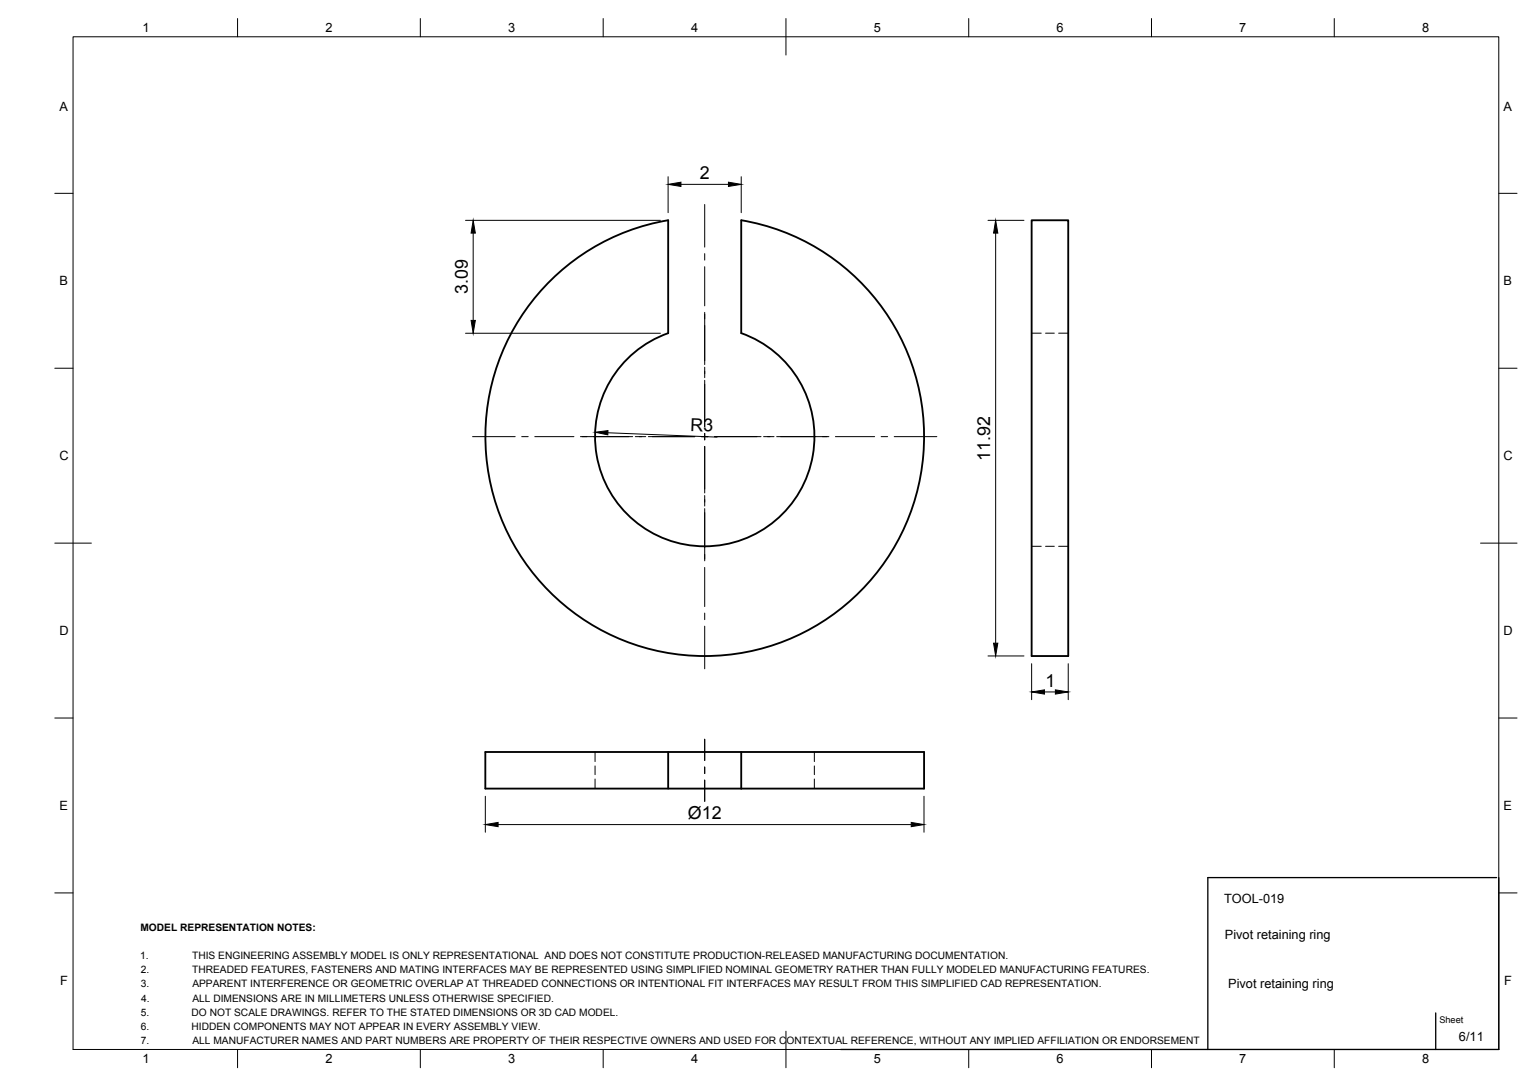
ISO-10303-21;
HEADER;
/* Generated by software containing ST-Developer
 * from STEP Tools, Inc. (www.steptools.com) 
 */

FILE_DESCRIPTION(
/* description */ (''),
/* implementation_level */ '2;1');

FILE_NAME(
/* name */ 'Pivot retaining ring.step',
/* time_stamp */ '2026-11-10T09:14:46-08:00',
/* author */ (''),
/* organization */ (''),
/* preprocessor_version */ 'ST-DEVELOPER v20.2',
/* originating_system */ 'Autodesk Translation Framework v15.17.0.0',
/* authorisation */ '');

FILE_SCHEMA (('AUTOMOTIVE_DESIGN { 1 0 10303 214 3 1 1 }'));
ENDSEC;

DATA;
#10=MECHANICAL_DESIGN_GEOMETRIC_PRESENTATION_REPRESENTATION('',(#561),#19471);
#541=SHAPE_REPRESENTATION_RELATIONSHIP('SRR','None',#19520,#551);
#551=ADVANCED_BREP_SHAPE_REPRESENTATION('',(#571),#19463);
#561=STYLED_ITEM('',(#19583),#571);
#571=MANIFOLD_SOLID_BREP('Body1',#7154);
#702=PLANE('',#7412);
#703=PLANE('',#7413);
#704=PLANE('',#7414);
#705=PLANE('',#7421);
#897=FACE_OUTER_BOUND('',#1325,.T.);
#898=FACE_OUTER_BOUND('',#1326,.T.);
#899=FACE_OUTER_BOUND('',#1327,.T.);
#900=FACE_OUTER_BOUND('',#1328,.T.);
#901=FACE_OUTER_BOUND('',#1329,.T.);
#902=FACE_OUTER_BOUND('',#1330,.T.);
#1325=EDGE_LOOP('',(#4925,#4926,#4927,#4928));
#1326=EDGE_LOOP('',(#4929,#4930,#4931,#4932));
#1327=EDGE_LOOP('',(#4933,#4934,#4935,#4936));
#1328=EDGE_LOOP('',(#4937,#4938,#4939,#4940));
#1329=EDGE_LOOP('',(#4941,#4942,#4943,#4944));
#1330=EDGE_LOOP('',(#4945,#4946,#4947,#4948));
#1843=LINE('',#9788,#2317);
#1844=LINE('',#9790,#2318);
#1845=LINE('',#9792,#2319);
#1846=LINE('',#9793,#2320);
#1847=LINE('',#9797,#2321);
#1848=LINE('',#9799,#2322);
#1849=LINE('',#9801,#2323);
#1850=LINE('',#9802,#2324);
#2317=VECTOR('',#8235,1.);
#2318=VECTOR('',#8236,1.);
#2319=VECTOR('',#8237,1.);
#2320=VECTOR('',#8238,1.);
#2321=VECTOR('',#8241,1.);
#2322=VECTOR('',#8242,1.);
#2323=VECTOR('',#8243,1.);
#2324=VECTOR('',#8244,1.);
#2715=CIRCLE('',#7415,0.6);
#2716=CIRCLE('',#7416,0.3);
#2717=CIRCLE('',#7418,0.3);
#2718=CIRCLE('',#7420,0.6);
#2971=VERTEX_POINT('',#9786);
#2972=VERTEX_POINT('',#9787);
#2973=VERTEX_POINT('',#9789);
#2974=VERTEX_POINT('',#9791);
#2975=VERTEX_POINT('',#9795);
#2976=VERTEX_POINT('',#9796);
#2977=VERTEX_POINT('',#9798);
#2978=VERTEX_POINT('',#9800);
#3703=EDGE_CURVE('',#2971,#2972,#1843,.T.);
#3704=EDGE_CURVE('',#2973,#2971,#1844,.T.);
#3705=EDGE_CURVE('',#2974,#2973,#1845,.T.);
#3706=EDGE_CURVE('',#2972,#2974,#1846,.T.);
#3707=EDGE_CURVE('',#2975,#2976,#1847,.T.);
#3708=EDGE_CURVE('',#2977,#2975,#1848,.T.);
#3709=EDGE_CURVE('',#2978,#2977,#1849,.T.);
#3710=EDGE_CURVE('',#2976,#2978,#1850,.T.);
#3711=EDGE_CURVE('',#2973,#2978,#2715,.T.);
#3712=EDGE_CURVE('',#2976,#2971,#2716,.T.);
#3713=EDGE_CURVE('',#2975,#2972,#2717,.T.);
#3714=EDGE_CURVE('',#2974,#2977,#2718,.T.);
#4925=ORIENTED_EDGE('',*,*,#3703,.F.);
#4926=ORIENTED_EDGE('',*,*,#3704,.F.);
#4927=ORIENTED_EDGE('',*,*,#3705,.F.);
#4928=ORIENTED_EDGE('',*,*,#3706,.F.);
#4929=ORIENTED_EDGE('',*,*,#3707,.F.);
#4930=ORIENTED_EDGE('',*,*,#3708,.F.);
#4931=ORIENTED_EDGE('',*,*,#3709,.F.);
#4932=ORIENTED_EDGE('',*,*,#3710,.F.);
#4933=ORIENTED_EDGE('',*,*,#3710,.T.);
#4934=ORIENTED_EDGE('',*,*,#3711,.F.);
#4935=ORIENTED_EDGE('',*,*,#3704,.T.);
#4936=ORIENTED_EDGE('',*,*,#3712,.F.);
#4937=ORIENTED_EDGE('',*,*,#3707,.T.);
#4938=ORIENTED_EDGE('',*,*,#3712,.T.);
#4939=ORIENTED_EDGE('',*,*,#3703,.T.);
#4940=ORIENTED_EDGE('',*,*,#3713,.F.);
#4941=ORIENTED_EDGE('',*,*,#3709,.T.);
#4942=ORIENTED_EDGE('',*,*,#3714,.F.);
#4943=ORIENTED_EDGE('',*,*,#3705,.T.);
#4944=ORIENTED_EDGE('',*,*,#3711,.T.);
#4945=ORIENTED_EDGE('',*,*,#3708,.T.);
#4946=ORIENTED_EDGE('',*,*,#3713,.T.);
#4947=ORIENTED_EDGE('',*,*,#3706,.T.);
#4948=ORIENTED_EDGE('',*,*,#3714,.T.);
#6625=CYLINDRICAL_SURFACE('',#7417,0.3);
#6626=CYLINDRICAL_SURFACE('',#7419,0.6);
#6819=ADVANCED_FACE('',(#897),#702,.F.);
#6820=ADVANCED_FACE('',(#898),#703,.F.);
#6821=ADVANCED_FACE('',(#899),#704,.F.);
#6822=ADVANCED_FACE('',(#900),#6625,.F.);
#6823=ADVANCED_FACE('',(#901),#6626,.T.);
#6824=ADVANCED_FACE('',(#902),#705,.T.);
#7154=CLOSED_SHELL('',(#6819,#6820,#6821,#6822,#6823,#6824));
#7411=AXIS2_PLACEMENT_3D('',#9784,#8231,#8232);
#7412=AXIS2_PLACEMENT_3D('',#9785,#8233,#8234);
#7413=AXIS2_PLACEMENT_3D('',#9794,#8239,#8240);
#7414=AXIS2_PLACEMENT_3D('',#9803,#8245,#8246);
#7415=AXIS2_PLACEMENT_3D('',#9804,#8247,#8248);
#7416=AXIS2_PLACEMENT_3D('',#9805,#8249,#8250);
#7417=AXIS2_PLACEMENT_3D('',#9806,#8251,#8252);
#7418=AXIS2_PLACEMENT_3D('',#9807,#8253,#8254);
#7419=AXIS2_PLACEMENT_3D('',#9808,#8255,#8256);
#7420=AXIS2_PLACEMENT_3D('',#9809,#8257,#8258);
#7421=AXIS2_PLACEMENT_3D('',#9810,#8259,#8260);
#8231=DIRECTION('axis',(0.,0.,1.));
#8232=DIRECTION('refdir',(1.,0.,0.));
#8233=DIRECTION('center_axis',(-1.,0.,0.));
#8234=DIRECTION('ref_axis',(0.,1.,0.));
#8235=DIRECTION('',(0.,0.,1.));
#8236=DIRECTION('',(0.,-1.,0.));
#8237=DIRECTION('',(0.,0.,-1.));
#8238=DIRECTION('',(0.,1.,0.));
#8239=DIRECTION('center_axis',(1.,0.,0.));
#8240=DIRECTION('ref_axis',(0.,-1.,0.));
#8241=DIRECTION('',(0.,0.,-1.));
#8242=DIRECTION('',(0.,-1.,0.));
#8243=DIRECTION('',(0.,0.,1.));
#8244=DIRECTION('',(0.,1.,0.));
#8245=DIRECTION('center_axis',(0.,0.,1.));
#8246=DIRECTION('ref_axis',(1.,0.,0.));
#8247=DIRECTION('center_axis',(0.,0.,1.));
#8248=DIRECTION('ref_axis',(1.,0.,0.));
#8249=DIRECTION('center_axis',(0.,0.,-1.));
#8250=DIRECTION('ref_axis',(1.,0.,0.));
#8251=DIRECTION('center_axis',(0.,0.,1.));
#8252=DIRECTION('ref_axis',(6.12323399573677E-17,-1.,0.));
#8253=DIRECTION('center_axis',(0.,0.,-1.));
#8254=DIRECTION('ref_axis',(1.,0.,0.));
#8255=DIRECTION('center_axis',(0.,0.,1.));
#8256=DIRECTION('ref_axis',(6.12323399573677E-17,-1.,0.));
#8257=DIRECTION('center_axis',(0.,0.,1.));
#8258=DIRECTION('ref_axis',(1.,0.,0.));
#8259=DIRECTION('center_axis',(0.,0.,1.));
#8260=DIRECTION('ref_axis',(1.,0.,0.));
#9784=CARTESIAN_POINT('',(0.,0.,0.));
#9785=CARTESIAN_POINT('Origin',(-0.1,0.,0.1));
#9786=CARTESIAN_POINT('',(-0.1,0.282842712474619,0.));
#9787=CARTESIAN_POINT('',(-0.1,0.282842712474619,0.1));
#9788=CARTESIAN_POINT('',(-0.1,0.282842712474619,0.));
#9789=CARTESIAN_POINT('',(-0.1,0.591607978309962,0.));
#9790=CARTESIAN_POINT('',(-0.1,0.,0.));
#9791=CARTESIAN_POINT('',(-0.1,0.591607978309962,0.1));
#9792=CARTESIAN_POINT('',(-0.1,0.591607978309962,0.));
#9793=CARTESIAN_POINT('',(-0.1,0.,0.1));
#9794=CARTESIAN_POINT('Origin',(0.1,1.2,0.1));
#9795=CARTESIAN_POINT('',(0.1,0.282842712474619,0.1));
#9796=CARTESIAN_POINT('',(0.1,0.282842712474619,0.));
#9797=CARTESIAN_POINT('',(0.1,0.282842712474619,0.));
#9798=CARTESIAN_POINT('',(0.1,0.591607978309962,0.1));
#9799=CARTESIAN_POINT('',(0.1,0.6,0.1));
#9800=CARTESIAN_POINT('',(0.1,0.591607978309962,0.));
#9801=CARTESIAN_POINT('',(0.1,0.591607978309962,0.));
#9802=CARTESIAN_POINT('',(0.1,0.6,0.));
#9803=CARTESIAN_POINT('Origin',(0.,0.,0.));
#9804=CARTESIAN_POINT('Origin',(0.,0.,0.));
#9805=CARTESIAN_POINT('Origin',(0.,0.,0.));
#9806=CARTESIAN_POINT('Origin',(0.,0.,0.));
#9807=CARTESIAN_POINT('Origin',(0.,0.,0.1));
#9808=CARTESIAN_POINT('Origin',(0.,0.,0.));
#9809=CARTESIAN_POINT('Origin',(0.,0.,0.1));
#9810=CARTESIAN_POINT('Origin',(0.,0.,0.1));
#19450=UNCERTAINTY_MEASURE_WITH_UNIT(LENGTH_MEASURE(0.001),#19472,
'DISTANCE_ACCURACY_VALUE',
'Maximum model space distance between geometric entities at asserted c
onnectivities');
#19458=UNCERTAINTY_MEASURE_WITH_UNIT(LENGTH_MEASURE(0.001),#19472,
'DISTANCE_ACCURACY_VALUE',
'Maximum model space distance between geometric entities at asserted c
onnectivities');
#19463=(
GEOMETRIC_REPRESENTATION_CONTEXT(3)
GLOBAL_UNCERTAINTY_ASSIGNED_CONTEXT((#19450))
GLOBAL_UNIT_ASSIGNED_CONTEXT((#19472,#19474,#19475))
REPRESENTATION_CONTEXT('','3D')
);
#19471=(
GEOMETRIC_REPRESENTATION_CONTEXT(3)
GLOBAL_UNCERTAINTY_ASSIGNED_CONTEXT((#19458))
GLOBAL_UNIT_ASSIGNED_CONTEXT((#19472,#19474,#19475))
REPRESENTATION_CONTEXT('','3D')
);
#19472=(
LENGTH_UNIT()
NAMED_UNIT(*)
SI_UNIT(.CENTI.,.METRE.)
);
#19474=(
NAMED_UNIT(*)
PLANE_ANGLE_UNIT()
SI_UNIT($,.RADIAN.)
);
#19475=(
NAMED_UNIT(*)
SI_UNIT($,.STERADIAN.)
SOLID_ANGLE_UNIT()
);
#19480=SHAPE_DEFINITION_REPRESENTATION(#19492,#19520);
#19492=PRODUCT_DEFINITION_SHAPE('',$,#19533);
#19520=SHAPE_REPRESENTATION('',(#7411),#19463);
#19528=PRODUCT_DEFINITION_CONTEXT('part definition',#19566,'design');
#19533=PRODUCT_DEFINITION('Pivot retaining ring','Pivot retaining ring',
#19545,#19528);
#19545=PRODUCT_DEFINITION_FORMATION('',$,#19572);
#19566=APPLICATION_CONTEXT(
'Core Data for Automotive Mechanical Design Process');
#19567=PRODUCT_CONTEXT('part definition',#19566,'mechanical');
#19572=PRODUCT('Pivot retaining ring','Pivot retaining ring',$,(#19567));
#19583=PRESENTATION_STYLE_ASSIGNMENT((#19591));
#19591=SURFACE_STYLE_USAGE(.BOTH.,#19599);
#19599=SURFACE_SIDE_STYLE('',(#19607));
#19607=SURFACE_STYLE_FILL_AREA(#19615);
#19615=FILL_AREA_STYLE('Dark gray',(#19623));
#19623=FILL_AREA_STYLE_COLOUR('Dark gray',#19631);
#19631=COLOUR_RGB('Dark gray',0.250980392156863,0.282352941176471,0.32156862745098);
ENDSEC;
END-ISO-10303-21;
